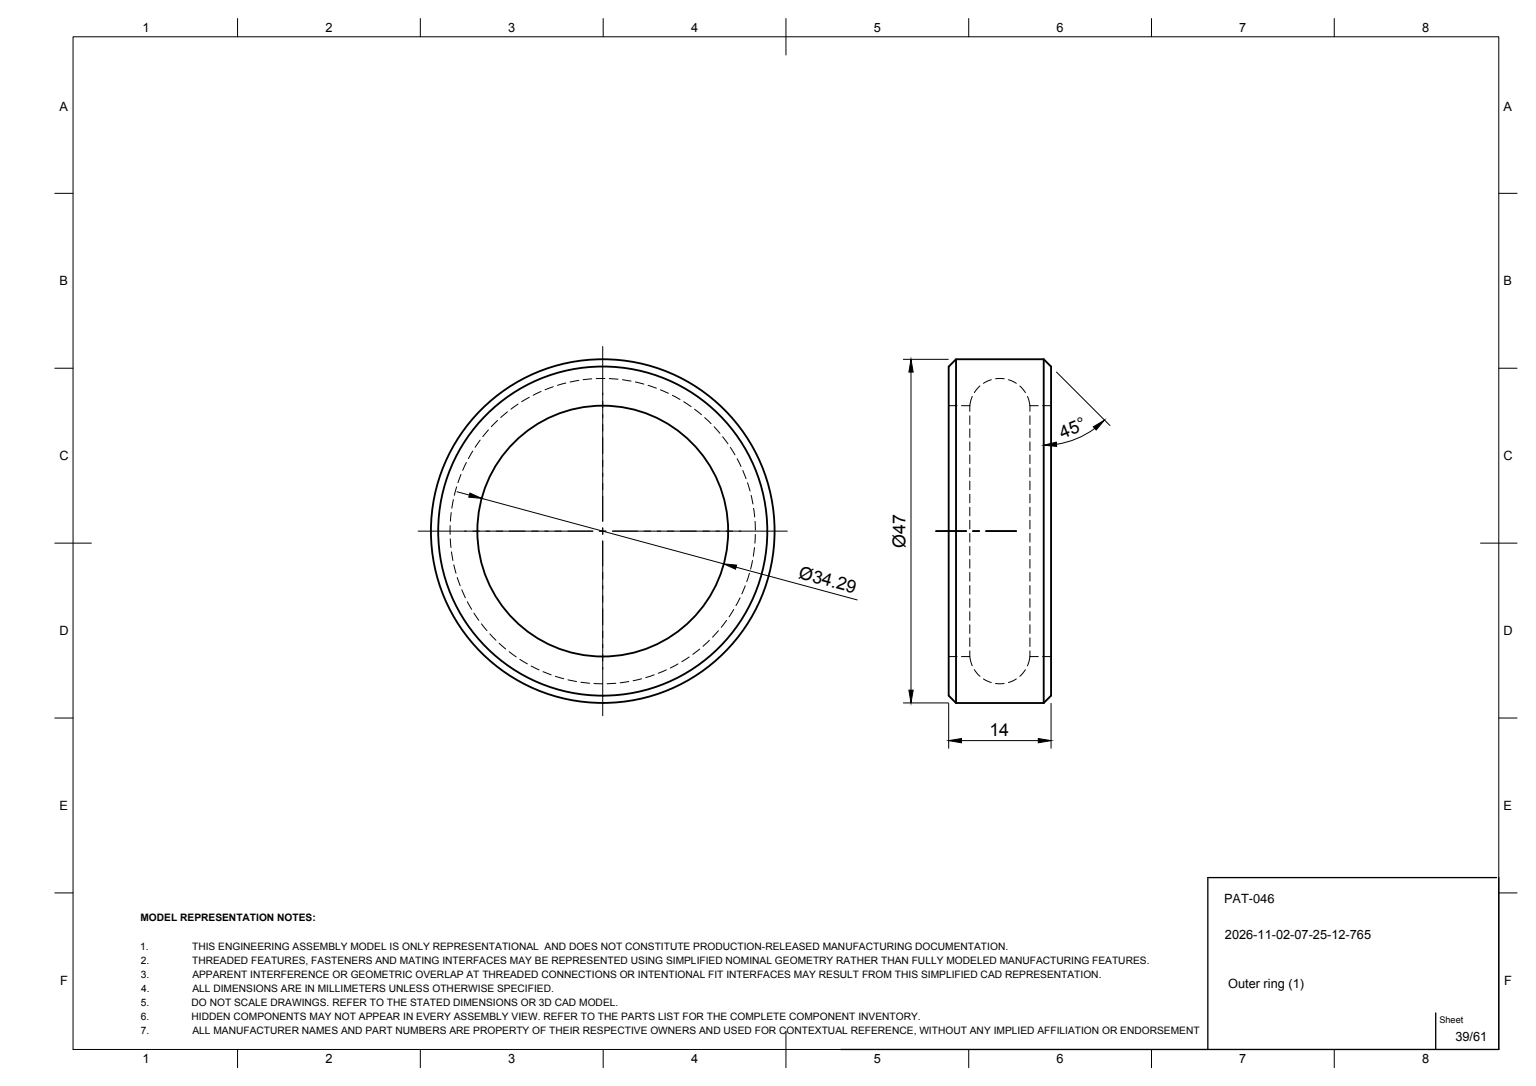
ISO-10303-21;
HEADER;
/* Generated by software containing ST-Developer
 * from STEP Tools, Inc. (www.steptools.com) 
 */

FILE_DESCRIPTION(
/* description */ ('Gear mesh backlash fixture'),
/* implementation_level */ '2;1');

FILE_NAME(
/* name */ 'Outer ring (1).step',
/* time_stamp */ '2026-10-28T03:26:00-07:00',
/* author */ (''),
/* organization */ (''),
/* preprocessor_version */ 'ST-DEVELOPER v20.2',
/* originating_system */ 'Autodesk Translation Framework v15.17.0.0',
/* authorisation */ '');

FILE_SCHEMA (('AUTOMOTIVE_DESIGN { 1 0 10303 214 3 1 1 }'));
ENDSEC;

DATA;
#10=MECHANICAL_DESIGN_GEOMETRIC_PRESENTATION_REPRESENTATION('',(#1052),#57900);
#774=CONICAL_SURFACE('',#14940,2.3,0.785398163397449);
#775=CONICAL_SURFACE('',#14944,2.3,0.785398163397449);
#783=TOROIDAL_SURFACE('',#14929,1.675,0.412776);
#945=SHAPE_REPRESENTATION_RELATIONSHIP('SRR','None',#58144,#995);
#995=ADVANCED_BREP_SHAPE_REPRESENTATION('',(#1115),#57877);
#1052=STYLED_ITEM('',(#58465),#1115);
#1115=MANIFOLD_SOLID_BREP('Body1',#13614);
#1284=FACE_BOUND('',#2961,.T.);
#1285=FACE_BOUND('',#2966,.T.);
#1534=PLANE('',#14937);
#1535=PLANE('',#14946);
#2052=FACE_OUTER_BOUND('',#2958,.T.);
#2053=FACE_OUTER_BOUND('',#2959,.T.);
#2054=FACE_OUTER_BOUND('',#2960,.T.);
#2055=FACE_OUTER_BOUND('',#2962,.T.);
#2056=FACE_OUTER_BOUND('',#2963,.T.);
#2057=FACE_OUTER_BOUND('',#2964,.T.);
#2058=FACE_OUTER_BOUND('',#2965,.T.);
#2059=FACE_OUTER_BOUND('',#2967,.T.);
#2958=EDGE_LOOP('',(#10507,#10508,#10509,#10510,#10511,#10512));
#2959=EDGE_LOOP('',(#10513,#10514,#10515,#10516,#10517));
#2960=EDGE_LOOP('',(#10518));
#2961=EDGE_LOOP('',(#10519));
#2962=EDGE_LOOP('',(#10520,#10521,#10522,#10523));
#2963=EDGE_LOOP('',(#10524,#10525,#10526,#10527));
#2964=EDGE_LOOP('',(#10528,#10529,#10530,#10531));
#2965=EDGE_LOOP('',(#10532));
#2966=EDGE_LOOP('',(#10533));
#2967=EDGE_LOOP('',(#10534,#10535,#10536,#10537,#10538));
#3868=LINE('',#21462,#4757);
#3869=LINE('',#21471,#4758);
#3870=LINE('',#21475,#4759);
#3871=LINE('',#21479,#4760);
#3872=LINE('',#21482,#4761);
#4757=VECTOR('',#17519,1.71469);
#4758=VECTOR('',#17530,2.3);
#4759=VECTOR('',#17535,2.35);
#4760=VECTOR('',#17540,2.3);
#4761=VECTOR('',#17545,1.71469);
#5521=CIRCLE('',#14930,1.71469);
#5522=CIRCLE('',#14931,1.71469);
#5523=CIRCLE('',#14932,0.412776);
#5524=CIRCLE('',#14933,1.71469);
#5525=CIRCLE('',#14934,1.71469);
#5526=CIRCLE('',#14936,1.71469);
#5527=CIRCLE('',#14938,2.25);
#5528=CIRCLE('',#14939,1.71469);
#5529=CIRCLE('',#14941,2.35);
#5530=CIRCLE('',#14943,2.35);
#5531=CIRCLE('',#14945,2.25);
#6324=VERTEX_POINT('',#21450);
#6325=VERTEX_POINT('',#21451);
#6326=VERTEX_POINT('',#21454);
#6327=VERTEX_POINT('',#21456);
#6328=VERTEX_POINT('',#21460);
#6329=VERTEX_POINT('',#21464);
#6330=VERTEX_POINT('',#21466);
#6331=VERTEX_POINT('',#21469);
#6332=VERTEX_POINT('',#21473);
#6333=VERTEX_POINT('',#21477);
#7840=EDGE_CURVE('',#6324,#6325,#5521,.T.);
#7841=EDGE_CURVE('',#6325,#6324,#5522,.T.);
#7842=EDGE_CURVE('',#6325,#6326,#5523,.T.);
#7843=EDGE_CURVE('',#6327,#6326,#5524,.T.);
#7844=EDGE_CURVE('',#6326,#6327,#5525,.T.);
#7845=EDGE_CURVE('',#6328,#6328,#5526,.T.);
#7846=EDGE_CURVE('',#6328,#6327,#3868,.T.);
#7847=EDGE_CURVE('',#6329,#6329,#5527,.T.);
#7848=EDGE_CURVE('',#6330,#6330,#5528,.T.);
#7849=EDGE_CURVE('',#6331,#6331,#5529,.T.);
#7850=EDGE_CURVE('',#6331,#6329,#3869,.T.);
#7851=EDGE_CURVE('',#6332,#6332,#5530,.T.);
#7852=EDGE_CURVE('',#6332,#6331,#3870,.T.);
#7853=EDGE_CURVE('',#6333,#6333,#5531,.T.);
#7854=EDGE_CURVE('',#6333,#6332,#3871,.T.);
#7855=EDGE_CURVE('',#6324,#6330,#3872,.T.);
#10507=ORIENTED_EDGE('',*,*,#7840,.F.);
#10508=ORIENTED_EDGE('',*,*,#7841,.F.);
#10509=ORIENTED_EDGE('',*,*,#7842,.T.);
#10510=ORIENTED_EDGE('',*,*,#7843,.F.);
#10511=ORIENTED_EDGE('',*,*,#7844,.F.);
#10512=ORIENTED_EDGE('',*,*,#7842,.F.);
#10513=ORIENTED_EDGE('',*,*,#7845,.T.);
#10514=ORIENTED_EDGE('',*,*,#7846,.T.);
#10515=ORIENTED_EDGE('',*,*,#7843,.T.);
#10516=ORIENTED_EDGE('',*,*,#7844,.T.);
#10517=ORIENTED_EDGE('',*,*,#7846,.F.);
#10518=ORIENTED_EDGE('',*,*,#7847,.F.);
#10519=ORIENTED_EDGE('',*,*,#7848,.T.);
#10520=ORIENTED_EDGE('',*,*,#7849,.F.);
#10521=ORIENTED_EDGE('',*,*,#7850,.T.);
#10522=ORIENTED_EDGE('',*,*,#7847,.T.);
#10523=ORIENTED_EDGE('',*,*,#7850,.F.);
#10524=ORIENTED_EDGE('',*,*,#7851,.F.);
#10525=ORIENTED_EDGE('',*,*,#7852,.T.);
#10526=ORIENTED_EDGE('',*,*,#7849,.T.);
#10527=ORIENTED_EDGE('',*,*,#7852,.F.);
#10528=ORIENTED_EDGE('',*,*,#7853,.F.);
#10529=ORIENTED_EDGE('',*,*,#7854,.T.);
#10530=ORIENTED_EDGE('',*,*,#7851,.T.);
#10531=ORIENTED_EDGE('',*,*,#7854,.F.);
#10532=ORIENTED_EDGE('',*,*,#7853,.T.);
#10533=ORIENTED_EDGE('',*,*,#7845,.F.);
#10534=ORIENTED_EDGE('',*,*,#7840,.T.);
#10535=ORIENTED_EDGE('',*,*,#7841,.T.);
#10536=ORIENTED_EDGE('',*,*,#7855,.T.);
#10537=ORIENTED_EDGE('',*,*,#7848,.F.);
#10538=ORIENTED_EDGE('',*,*,#7855,.F.);
#12707=CYLINDRICAL_SURFACE('',#14935,1.71469);
#12708=CYLINDRICAL_SURFACE('',#14942,2.35);
#12709=CYLINDRICAL_SURFACE('',#14947,1.71469);
#13169=ADVANCED_FACE('',(#2052),#783,.F.);
#13170=ADVANCED_FACE('',(#2053),#12707,.F.);
#13171=ADVANCED_FACE('',(#2054,#1284),#1534,.T.);
#13172=ADVANCED_FACE('',(#2055),#774,.T.);
#13173=ADVANCED_FACE('',(#2056),#12708,.T.);
#13174=ADVANCED_FACE('',(#2057),#775,.T.);
#13175=ADVANCED_FACE('',(#2058,#1285),#1535,.T.);
#13176=ADVANCED_FACE('',(#2059),#12709,.F.);
#13614=CLOSED_SHELL('',(#13169,#13170,#13171,#13172,#13173,#13174,#13175,
#13176));
#14928=AXIS2_PLACEMENT_3D('',#21448,#17501,#17502);
#14929=AXIS2_PLACEMENT_3D('',#21449,#17503,#17504);
#14930=AXIS2_PLACEMENT_3D('',#21452,#17505,#17506);
#14931=AXIS2_PLACEMENT_3D('',#21453,#17507,#17508);
#14932=AXIS2_PLACEMENT_3D('',#21455,#17509,#17510);
#14933=AXIS2_PLACEMENT_3D('',#21457,#17511,#17512);
#14934=AXIS2_PLACEMENT_3D('',#21458,#17513,#17514);
#14935=AXIS2_PLACEMENT_3D('',#21459,#17515,#17516);
#14936=AXIS2_PLACEMENT_3D('',#21461,#17517,#17518);
#14937=AXIS2_PLACEMENT_3D('',#21463,#17520,#17521);
#14938=AXIS2_PLACEMENT_3D('',#21465,#17522,#17523);
#14939=AXIS2_PLACEMENT_3D('',#21467,#17524,#17525);
#14940=AXIS2_PLACEMENT_3D('',#21468,#17526,#17527);
#14941=AXIS2_PLACEMENT_3D('',#21470,#17528,#17529);
#14942=AXIS2_PLACEMENT_3D('',#21472,#17531,#17532);
#14943=AXIS2_PLACEMENT_3D('',#21474,#17533,#17534);
#14944=AXIS2_PLACEMENT_3D('',#21476,#17536,#17537);
#14945=AXIS2_PLACEMENT_3D('',#21478,#17538,#17539);
#14946=AXIS2_PLACEMENT_3D('',#21480,#17541,#17542);
#14947=AXIS2_PLACEMENT_3D('',#21481,#17543,#17544);
#17501=DIRECTION('axis',(0.,0.,1.));
#17502=DIRECTION('refdir',(1.,0.,0.));
#17503=DIRECTION('center_axis',(0.,-1.,0.));
#17504=DIRECTION('ref_axis',(0.,0.,-1.));
#17505=DIRECTION('center_axis',(0.,-1.,0.));
#17506=DIRECTION('ref_axis',(1.,0.,0.));
#17507=DIRECTION('center_axis',(0.,-1.,0.));
#17508=DIRECTION('ref_axis',(1.,0.,0.));
#17509=DIRECTION('center_axis',(1.,0.,1.22464679914735E-16));
#17510=DIRECTION('ref_axis',(-1.22464679914735E-16,0.,1.));
#17511=DIRECTION('center_axis',(0.,1.,0.));
#17512=DIRECTION('ref_axis',(1.,0.,0.));
#17513=DIRECTION('center_axis',(0.,1.,0.));
#17514=DIRECTION('ref_axis',(1.,0.,0.));
#17515=DIRECTION('center_axis',(0.,-1.,0.));
#17516=DIRECTION('ref_axis',(1.,0.,0.));
#17517=DIRECTION('center_axis',(0.,-1.,0.));
#17518=DIRECTION('ref_axis',(1.,0.,0.));
#17519=DIRECTION('',(0.,1.,0.));
#17520=DIRECTION('center_axis',(0.,1.,0.));
#17521=DIRECTION('ref_axis',(0.,0.,1.));
#17522=DIRECTION('center_axis',(0.,-1.,0.));
#17523=DIRECTION('ref_axis',(1.,0.,0.));
#17524=DIRECTION('center_axis',(0.,-1.,0.));
#17525=DIRECTION('ref_axis',(1.,0.,0.));
#17526=DIRECTION('center_axis',(0.,-1.,0.));
#17527=DIRECTION('ref_axis',(1.,0.,0.));
#17528=DIRECTION('center_axis',(0.,-1.,0.));
#17529=DIRECTION('ref_axis',(1.,0.,0.));
#17530=DIRECTION('',(0.707106781186548,0.707106781186547,8.65956056235494E-17));
#17531=DIRECTION('center_axis',(0.,-1.,0.));
#17532=DIRECTION('ref_axis',(1.,0.,0.));
#17533=DIRECTION('center_axis',(0.,-1.,0.));
#17534=DIRECTION('ref_axis',(1.,0.,0.));
#17535=DIRECTION('',(0.,1.,0.));
#17536=DIRECTION('center_axis',(0.,1.,0.));
#17537=DIRECTION('ref_axis',(1.,0.,0.));
#17538=DIRECTION('center_axis',(0.,-1.,0.));
#17539=DIRECTION('ref_axis',(1.,0.,0.));
#17540=DIRECTION('',(-0.707106781186548,0.707106781186547,-8.65956056235494E-17));
#17541=DIRECTION('center_axis',(0.,-1.,0.));
#17542=DIRECTION('ref_axis',(0.,0.,-1.));
#17543=DIRECTION('center_axis',(0.,-1.,0.));
#17544=DIRECTION('ref_axis',(1.,0.,0.));
#17545=DIRECTION('',(0.,1.,0.));
#21448=CARTESIAN_POINT('',(0.,0.,0.));
#21449=CARTESIAN_POINT('Origin',(0.,0.,0.));
#21450=CARTESIAN_POINT('',(-1.71469,0.410863395882378,-2.09988962002998E-16));
#21451=CARTESIAN_POINT('',(-2.09988962002998E-16,0.410863395882378,1.71469));
#21452=CARTESIAN_POINT('Origin',(0.,0.410863395882378,0.));
#21453=CARTESIAN_POINT('Origin',(0.,0.410863395882378,0.));
#21454=CARTESIAN_POINT('',(-2.09988962002998E-16,-0.410863395882378,1.71469));
#21455=CARTESIAN_POINT('Origin',(-2.05128338857182E-16,0.,1.675));
#21456=CARTESIAN_POINT('',(-1.71469,-0.410863395882378,2.09988962002998E-16));
#21457=CARTESIAN_POINT('Origin',(0.,-0.410863395882378,0.));
#21458=CARTESIAN_POINT('Origin',(0.,-0.410863395882378,0.));
#21459=CARTESIAN_POINT('Origin',(0.,0.,0.));
#21460=CARTESIAN_POINT('',(-1.71469,-0.7,-2.09988962002998E-16));
#21461=CARTESIAN_POINT('Origin',(0.,-0.7,0.));
#21462=CARTESIAN_POINT('',(-1.71469,0.,-2.09988962002998E-16));
#21463=CARTESIAN_POINT('Origin',(2.25,0.7,0.));
#21464=CARTESIAN_POINT('',(-2.25,0.7,-2.75545529808154E-16));
#21465=CARTESIAN_POINT('Origin',(0.,0.7,0.));
#21466=CARTESIAN_POINT('',(-1.71469,0.7,-2.09988962002998E-16));
#21467=CARTESIAN_POINT('Origin',(0.,0.7,0.));
#21468=CARTESIAN_POINT('Origin',(0.,0.65,0.));
#21469=CARTESIAN_POINT('',(-2.35,0.6,-2.87791997799628E-16));
#21470=CARTESIAN_POINT('Origin',(0.,0.6,0.));
#21471=CARTESIAN_POINT('',(-2.3,0.65,-2.81668763803891E-16));
#21472=CARTESIAN_POINT('Origin',(0.,0.,0.));
#21473=CARTESIAN_POINT('',(-2.35,-0.6,-2.87791997799628E-16));
#21474=CARTESIAN_POINT('Origin',(0.,-0.6,0.));
#21475=CARTESIAN_POINT('',(-2.35,0.,-2.87791997799628E-16));
#21476=CARTESIAN_POINT('Origin',(0.,-0.65,0.));
#21477=CARTESIAN_POINT('',(-2.25,-0.7,-2.75545529808154E-16));
#21478=CARTESIAN_POINT('Origin',(0.,-0.7,0.));
#21479=CARTESIAN_POINT('',(-2.3,-0.65,-2.81668763803891E-16));
#21480=CARTESIAN_POINT('Origin',(1.71469,-0.7,0.));
#21481=CARTESIAN_POINT('Origin',(0.,0.,0.));
#21482=CARTESIAN_POINT('',(-1.71469,0.,-2.09988962002998E-16));
#57818=UNCERTAINTY_MEASURE_WITH_UNIT(LENGTH_MEASURE(0.001),#57901,
'DISTANCE_ACCURACY_VALUE',
'Maximum model space distance between geometric entities at asserted c
onnectivities');
#57841=UNCERTAINTY_MEASURE_WITH_UNIT(LENGTH_MEASURE(0.001),#57901,
'DISTANCE_ACCURACY_VALUE',
'Maximum model space distance between geometric entities at asserted c
onnectivities');
#57877=(
GEOMETRIC_REPRESENTATION_CONTEXT(3)
GLOBAL_UNCERTAINTY_ASSIGNED_CONTEXT((#57818))
GLOBAL_UNIT_ASSIGNED_CONTEXT((#57901,#57903,#57904))
REPRESENTATION_CONTEXT('','3D')
);
#57900=(
GEOMETRIC_REPRESENTATION_CONTEXT(3)
GLOBAL_UNCERTAINTY_ASSIGNED_CONTEXT((#57841))
GLOBAL_UNIT_ASSIGNED_CONTEXT((#57901,#57903,#57904))
REPRESENTATION_CONTEXT('','3D')
);
#57901=(
LENGTH_UNIT()
NAMED_UNIT(*)
SI_UNIT(.CENTI.,.METRE.)
);
#57903=(
NAMED_UNIT(*)
PLANE_ANGLE_UNIT()
SI_UNIT($,.RADIAN.)
);
#57904=(
NAMED_UNIT(*)
SI_UNIT($,.STERADIAN.)
SOLID_ANGLE_UNIT()
);
#57940=SHAPE_DEFINITION_REPRESENTATION(#58006,#58144);
#58006=PRODUCT_DEFINITION_SHAPE('',$,#58203);
#58144=SHAPE_REPRESENTATION('',(#14928),#57877);
#58167=PRODUCT_DEFINITION_CONTEXT('part definition',#58343,'design');
#58203=PRODUCT_DEFINITION('Outer ring (1)','Outer ring (1)',#58261,#58167);
#58261=PRODUCT_DEFINITION_FORMATION('',$,#58380);
#58343=APPLICATION_CONTEXT(
'Core Data for Automotive Mechanical Design Process');
#58344=PRODUCT_CONTEXT('part definition',#58343,'mechanical');
#58380=PRODUCT('Outer ring (1)','Outer ring (1)','Outer ring (1)',(#58344));
#58459=COLOUR_RGB('Grey',0.48,0.52,0.57);
#58460=FILL_AREA_STYLE_COLOUR('',#58459);
#58461=FILL_AREA_STYLE('',(#58460));
#58462=SURFACE_STYLE_FILL_AREA(#58461);
#58463=SURFACE_SIDE_STYLE('',(#58462));
#58464=SURFACE_STYLE_USAGE(.BOTH.,#58463);
#58465=PRESENTATION_STYLE_ASSIGNMENT((#58464));
ENDSEC;
END-ISO-10303-21;
